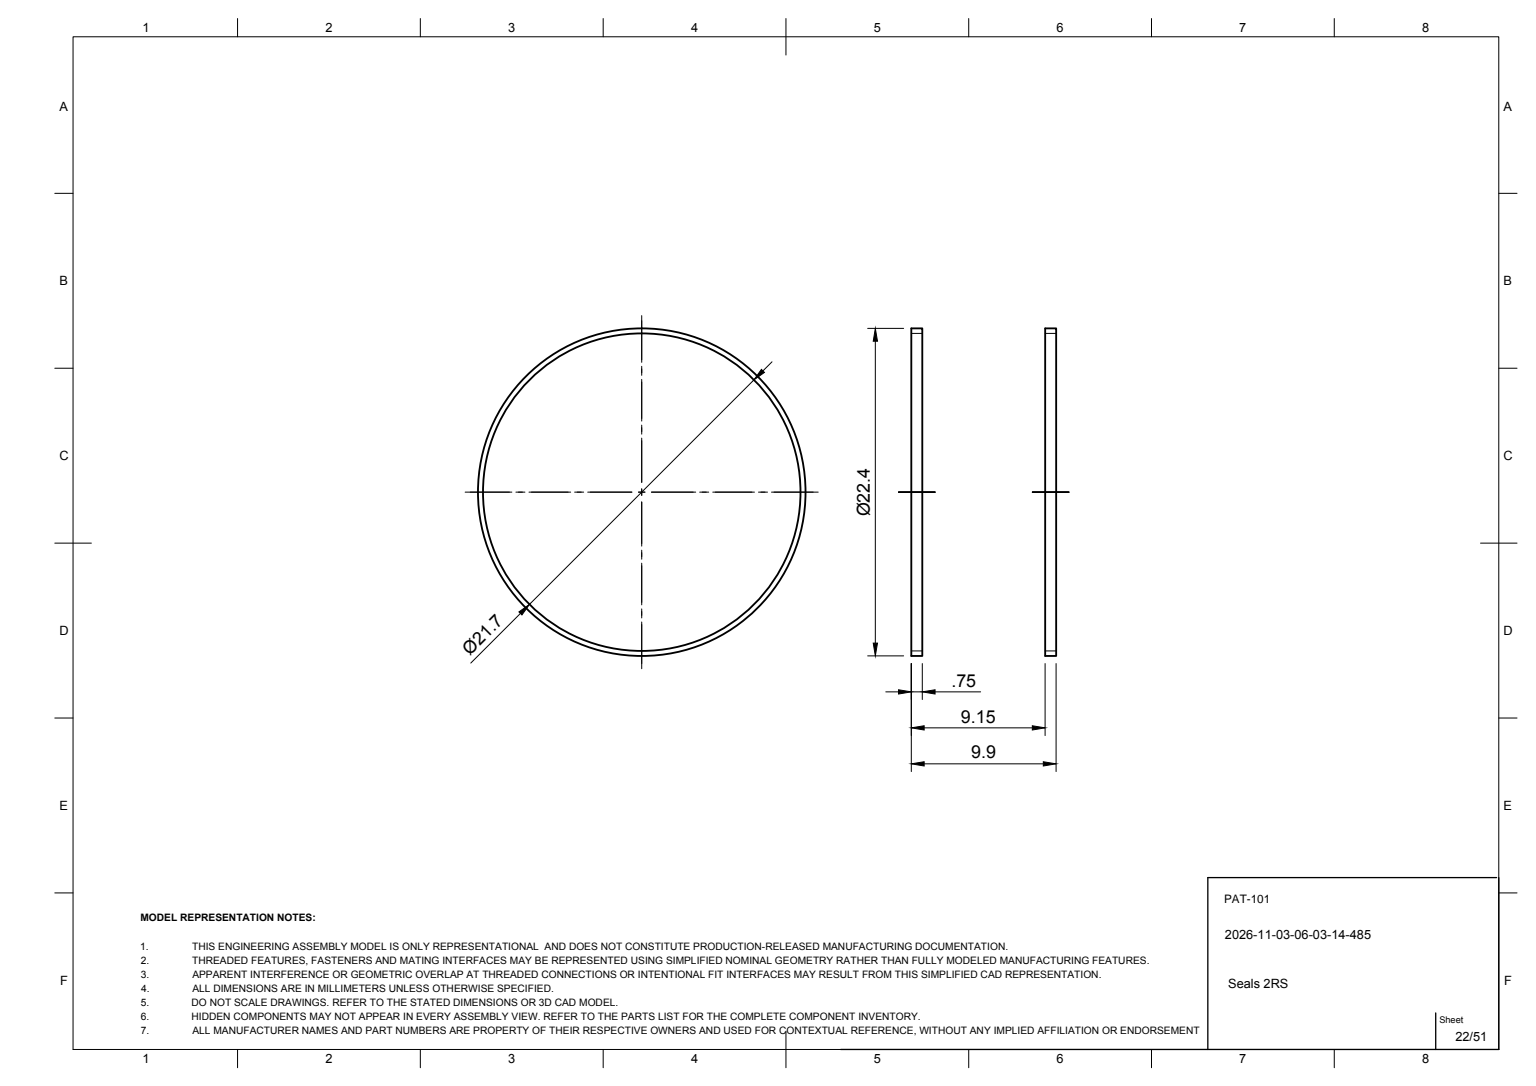
ISO-10303-21;
HEADER;
/* Generated by software containing ST-Developer
 * from STEP Tools, Inc. (www.steptools.com) 
 */

FILE_DESCRIPTION(
/* description */ ('Spur gear reduction stage 2-1 on bearing plates'),
/* implementation_level */ '2;1');

FILE_NAME(
/* name */ 'Seals 2RS.step',
/* time_stamp */ '2026-10-28T03:22:07-07:00',
/* author */ (''),
/* organization */ (''),
/* preprocessor_version */ 'ST-DEVELOPER v20.2',
/* originating_system */ 'Autodesk Translation Framework v15.17.0.0',
/* authorisation */ '');

FILE_SCHEMA (('AUTOMOTIVE_DESIGN { 1 0 10303 214 3 1 1 }'));
ENDSEC;

DATA;
#10=MECHANICAL_DESIGN_GEOMETRIC_PRESENTATION_REPRESENTATION('',(#970,#971),#53909);
#878=SHAPE_REPRESENTATION_RELATIONSHIP('SRR','None',#54106,#921);
#921=ADVANCED_BREP_SHAPE_REPRESENTATION('',(#1026,#1027),#53880);
#970=STYLED_ITEM('',(#54397),#1026);
#971=STYLED_ITEM('',(#54397),#1027);
#1026=MANIFOLD_SOLID_BREP('Body1',#11296);
#1027=MANIFOLD_SOLID_BREP('Body2',#11297);
#1183=FACE_BOUND('',#2479,.T.);
#1184=FACE_BOUND('',#2482,.T.);
#1185=FACE_BOUND('',#2485,.T.);
#1186=FACE_BOUND('',#2488,.T.);
#1326=PLANE('',#12260);
#1327=PLANE('',#12265);
#1328=PLANE('',#12268);
#1329=PLANE('',#12273);
#1707=FACE_OUTER_BOUND('',#2478,.T.);
#1708=FACE_OUTER_BOUND('',#2480,.T.);
#1709=FACE_OUTER_BOUND('',#2481,.T.);
#1710=FACE_OUTER_BOUND('',#2483,.T.);
#1711=FACE_OUTER_BOUND('',#2484,.T.);
#1712=FACE_OUTER_BOUND('',#2486,.T.);
#1713=FACE_OUTER_BOUND('',#2487,.T.);
#1714=FACE_OUTER_BOUND('',#2489,.T.);
#2478=EDGE_LOOP('',(#8182));
#2479=EDGE_LOOP('',(#8183));
#2480=EDGE_LOOP('',(#8184,#8185,#8186,#8187));
#2481=EDGE_LOOP('',(#8188));
#2482=EDGE_LOOP('',(#8189));
#2483=EDGE_LOOP('',(#8190,#8191,#8192,#8193));
#2484=EDGE_LOOP('',(#8194));
#2485=EDGE_LOOP('',(#8195));
#2486=EDGE_LOOP('',(#8196,#8197,#8198,#8199));
#2487=EDGE_LOOP('',(#8200));
#2488=EDGE_LOOP('',(#8201));
#2489=EDGE_LOOP('',(#8202,#8203,#8204,#8205));
#3149=LINE('',#17199,#3790);
#3150=LINE('',#17204,#3791);
#3151=LINE('',#17213,#3792);
#3152=LINE('',#17218,#3793);
#3790=VECTOR('',#14072,1.119765);
#3791=VECTOR('',#14079,1.085235);
#3792=VECTOR('',#14090,1.119765);
#3793=VECTOR('',#14097,1.085235);
#4488=CIRCLE('',#12261,1.119765);
#4489=CIRCLE('',#12262,1.085235);
#4490=CIRCLE('',#12264,1.119765);
#4491=CIRCLE('',#12266,1.085235);
#4492=CIRCLE('',#12269,1.119765);
#4493=CIRCLE('',#12270,1.085235);
#4494=CIRCLE('',#12272,1.119765);
#4495=CIRCLE('',#12274,1.085235);
#5066=VERTEX_POINT('',#17192);
#5067=VERTEX_POINT('',#17194);
#5068=VERTEX_POINT('',#17197);
#5069=VERTEX_POINT('',#17201);
#5070=VERTEX_POINT('',#17206);
#5071=VERTEX_POINT('',#17208);
#5072=VERTEX_POINT('',#17211);
#5073=VERTEX_POINT('',#17215);
#6233=EDGE_CURVE('',#5066,#5066,#4488,.T.);
#6234=EDGE_CURVE('',#5067,#5067,#4489,.T.);
#6235=EDGE_CURVE('',#5068,#5068,#4490,.T.);
#6236=EDGE_CURVE('',#5068,#5066,#3149,.T.);
#6237=EDGE_CURVE('',#5069,#5069,#4491,.T.);
#6238=EDGE_CURVE('',#5069,#5067,#3150,.T.);
#6239=EDGE_CURVE('',#5070,#5070,#4492,.T.);
#6240=EDGE_CURVE('',#5071,#5071,#4493,.T.);
#6241=EDGE_CURVE('',#5072,#5072,#4494,.T.);
#6242=EDGE_CURVE('',#5072,#5070,#3151,.T.);
#6243=EDGE_CURVE('',#5073,#5073,#4495,.T.);
#6244=EDGE_CURVE('',#5073,#5071,#3152,.T.);
#8182=ORIENTED_EDGE('',*,*,#6233,.F.);
#8183=ORIENTED_EDGE('',*,*,#6234,.T.);
#8184=ORIENTED_EDGE('',*,*,#6235,.F.);
#8185=ORIENTED_EDGE('',*,*,#6236,.T.);
#8186=ORIENTED_EDGE('',*,*,#6233,.T.);
#8187=ORIENTED_EDGE('',*,*,#6236,.F.);
#8188=ORIENTED_EDGE('',*,*,#6235,.T.);
#8189=ORIENTED_EDGE('',*,*,#6237,.F.);
#8190=ORIENTED_EDGE('',*,*,#6237,.T.);
#8191=ORIENTED_EDGE('',*,*,#6238,.T.);
#8192=ORIENTED_EDGE('',*,*,#6234,.F.);
#8193=ORIENTED_EDGE('',*,*,#6238,.F.);
#8194=ORIENTED_EDGE('',*,*,#6239,.F.);
#8195=ORIENTED_EDGE('',*,*,#6240,.T.);
#8196=ORIENTED_EDGE('',*,*,#6241,.F.);
#8197=ORIENTED_EDGE('',*,*,#6242,.T.);
#8198=ORIENTED_EDGE('',*,*,#6239,.T.);
#8199=ORIENTED_EDGE('',*,*,#6242,.F.);
#8200=ORIENTED_EDGE('',*,*,#6241,.T.);
#8201=ORIENTED_EDGE('',*,*,#6243,.F.);
#8202=ORIENTED_EDGE('',*,*,#6243,.T.);
#8203=ORIENTED_EDGE('',*,*,#6244,.T.);
#8204=ORIENTED_EDGE('',*,*,#6240,.F.);
#8205=ORIENTED_EDGE('',*,*,#6244,.F.);
#10508=CYLINDRICAL_SURFACE('',#12263,1.119765);
#10509=CYLINDRICAL_SURFACE('',#12267,1.085235);
#10510=CYLINDRICAL_SURFACE('',#12271,1.119765);
#10511=CYLINDRICAL_SURFACE('',#12275,1.085235);
#10827=ADVANCED_FACE('',(#1707,#1183),#1326,.T.);
#10828=ADVANCED_FACE('',(#1708),#10508,.T.);
#10829=ADVANCED_FACE('',(#1709,#1184),#1327,.T.);
#10830=ADVANCED_FACE('',(#1710),#10509,.F.);
#10831=ADVANCED_FACE('',(#1711,#1185),#1328,.T.);
#10832=ADVANCED_FACE('',(#1712),#10510,.T.);
#10833=ADVANCED_FACE('',(#1713,#1186),#1329,.T.);
#10834=ADVANCED_FACE('',(#1714),#10511,.F.);
#11296=CLOSED_SHELL('',(#10827,#10828,#10829,#10830));
#11297=CLOSED_SHELL('',(#10831,#10832,#10833,#10834));
#12259=AXIS2_PLACEMENT_3D('',#17190,#14060,#14061);
#12260=AXIS2_PLACEMENT_3D('',#17191,#14062,#14063);
#12261=AXIS2_PLACEMENT_3D('',#17193,#14064,#14065);
#12262=AXIS2_PLACEMENT_3D('',#17195,#14066,#14067);
#12263=AXIS2_PLACEMENT_3D('',#17196,#14068,#14069);
#12264=AXIS2_PLACEMENT_3D('',#17198,#14070,#14071);
#12265=AXIS2_PLACEMENT_3D('',#17200,#14073,#14074);
#12266=AXIS2_PLACEMENT_3D('',#17202,#14075,#14076);
#12267=AXIS2_PLACEMENT_3D('',#17203,#14077,#14078);
#12268=AXIS2_PLACEMENT_3D('',#17205,#14080,#14081);
#12269=AXIS2_PLACEMENT_3D('',#17207,#14082,#14083);
#12270=AXIS2_PLACEMENT_3D('',#17209,#14084,#14085);
#12271=AXIS2_PLACEMENT_3D('',#17210,#14086,#14087);
#12272=AXIS2_PLACEMENT_3D('',#17212,#14088,#14089);
#12273=AXIS2_PLACEMENT_3D('',#17214,#14091,#14092);
#12274=AXIS2_PLACEMENT_3D('',#17216,#14093,#14094);
#12275=AXIS2_PLACEMENT_3D('',#17217,#14095,#14096);
#14060=DIRECTION('axis',(0.,0.,1.));
#14061=DIRECTION('refdir',(1.,0.,0.));
#14062=DIRECTION('center_axis',(0.,1.,0.));
#14063=DIRECTION('ref_axis',(0.,0.,1.));
#14064=DIRECTION('center_axis',(0.,-1.,0.));
#14065=DIRECTION('ref_axis',(1.,0.,0.));
#14066=DIRECTION('center_axis',(0.,-1.,0.));
#14067=DIRECTION('ref_axis',(1.,0.,0.));
#14068=DIRECTION('center_axis',(0.,-1.,0.));
#14069=DIRECTION('ref_axis',(1.,0.,0.));
#14070=DIRECTION('center_axis',(0.,-1.,0.));
#14071=DIRECTION('ref_axis',(1.,0.,0.));
#14072=DIRECTION('',(0.,1.,0.));
#14073=DIRECTION('center_axis',(0.,-1.,0.));
#14074=DIRECTION('ref_axis',(0.,0.,-1.));
#14075=DIRECTION('center_axis',(0.,-1.,0.));
#14076=DIRECTION('ref_axis',(1.,0.,0.));
#14077=DIRECTION('center_axis',(0.,-1.,0.));
#14078=DIRECTION('ref_axis',(1.,0.,0.));
#14079=DIRECTION('',(0.,1.,0.));
#14080=DIRECTION('center_axis',(0.,1.,0.));
#14081=DIRECTION('ref_axis',(0.,0.,1.));
#14082=DIRECTION('center_axis',(0.,-1.,0.));
#14083=DIRECTION('ref_axis',(1.,0.,0.));
#14084=DIRECTION('center_axis',(0.,-1.,0.));
#14085=DIRECTION('ref_axis',(1.,0.,0.));
#14086=DIRECTION('center_axis',(0.,-1.,0.));
#14087=DIRECTION('ref_axis',(1.,0.,0.));
#14088=DIRECTION('center_axis',(0.,-1.,0.));
#14089=DIRECTION('ref_axis',(1.,0.,0.));
#14090=DIRECTION('',(0.,1.,0.));
#14091=DIRECTION('center_axis',(0.,-1.,0.));
#14092=DIRECTION('ref_axis',(0.,0.,-1.));
#14093=DIRECTION('center_axis',(0.,-1.,0.));
#14094=DIRECTION('ref_axis',(1.,0.,0.));
#14095=DIRECTION('center_axis',(0.,-1.,0.));
#14096=DIRECTION('ref_axis',(1.,0.,0.));
#14097=DIRECTION('',(0.,1.,0.));
#17190=CARTESIAN_POINT('',(0.,0.,0.));
#17191=CARTESIAN_POINT('Origin',(1.119765,0.495,0.));
#17192=CARTESIAN_POINT('',(-1.119765,0.495,-1.37131662304724E-16));
#17193=CARTESIAN_POINT('Origin',(0.,0.495,0.));
#17194=CARTESIAN_POINT('',(-1.085235,0.495,-1.32902956907268E-16));
#17195=CARTESIAN_POINT('Origin',(0.,0.495,0.));
#17196=CARTESIAN_POINT('Origin',(0.,0.4575,0.));
#17197=CARTESIAN_POINT('',(-1.119765,0.42,-1.37131662304724E-16));
#17198=CARTESIAN_POINT('Origin',(0.,0.42,0.));
#17199=CARTESIAN_POINT('',(-1.119765,0.4575,-1.37131662304724E-16));
#17200=CARTESIAN_POINT('Origin',(1.085235,0.42,0.));
#17201=CARTESIAN_POINT('',(-1.085235,0.42,-1.32902956907268E-16));
#17202=CARTESIAN_POINT('Origin',(0.,0.42,0.));
#17203=CARTESIAN_POINT('Origin',(0.,0.4575,0.));
#17204=CARTESIAN_POINT('',(-1.085235,0.4575,-1.32902956907268E-16));
#17205=CARTESIAN_POINT('Origin',(1.119765,-0.42,0.));
#17206=CARTESIAN_POINT('',(-1.119765,-0.42,-1.37131662304724E-16));
#17207=CARTESIAN_POINT('Origin',(0.,-0.42,0.));
#17208=CARTESIAN_POINT('',(-1.085235,-0.42,-1.32902956907268E-16));
#17209=CARTESIAN_POINT('Origin',(0.,-0.42,0.));
#17210=CARTESIAN_POINT('Origin',(0.,-0.4575,0.));
#17211=CARTESIAN_POINT('',(-1.119765,-0.495,-1.37131662304724E-16));
#17212=CARTESIAN_POINT('Origin',(0.,-0.495,0.));
#17213=CARTESIAN_POINT('',(-1.119765,-0.4575,-1.37131662304724E-16));
#17214=CARTESIAN_POINT('Origin',(1.085235,-0.495,0.));
#17215=CARTESIAN_POINT('',(-1.085235,-0.495,-1.32902956907268E-16));
#17216=CARTESIAN_POINT('Origin',(0.,-0.495,0.));
#17217=CARTESIAN_POINT('Origin',(0.,-0.4575,0.));
#17218=CARTESIAN_POINT('',(-1.085235,-0.4575,-1.32902956907268E-16));
#53830=UNCERTAINTY_MEASURE_WITH_UNIT(LENGTH_MEASURE(0.001),#53910,
'DISTANCE_ACCURACY_VALUE',
'Maximum model space distance between geometric entities at asserted c
onnectivities');
#53859=UNCERTAINTY_MEASURE_WITH_UNIT(LENGTH_MEASURE(0.001),#53910,
'DISTANCE_ACCURACY_VALUE',
'Maximum model space distance between geometric entities at asserted c
onnectivities');
#53880=(
GEOMETRIC_REPRESENTATION_CONTEXT(3)
GLOBAL_UNCERTAINTY_ASSIGNED_CONTEXT((#53830))
GLOBAL_UNIT_ASSIGNED_CONTEXT((#53910,#53912,#53913))
REPRESENTATION_CONTEXT('','3D')
);
#53909=(
GEOMETRIC_REPRESENTATION_CONTEXT(3)
GLOBAL_UNCERTAINTY_ASSIGNED_CONTEXT((#53859))
GLOBAL_UNIT_ASSIGNED_CONTEXT((#53910,#53912,#53913))
REPRESENTATION_CONTEXT('','3D')
);
#53910=(
LENGTH_UNIT()
NAMED_UNIT(*)
SI_UNIT(.CENTI.,.METRE.)
);
#53912=(
NAMED_UNIT(*)
PLANE_ANGLE_UNIT()
SI_UNIT($,.RADIAN.)
);
#53913=(
NAMED_UNIT(*)
SI_UNIT($,.STERADIAN.)
SOLID_ANGLE_UNIT()
);
#53934=SHAPE_DEFINITION_REPRESENTATION(#53983,#54106);
#53983=PRODUCT_DEFINITION_SHAPE('',$,#54156);
#54106=SHAPE_REPRESENTATION('',(#12259),#53880);
#54135=PRODUCT_DEFINITION_CONTEXT('part definition',#54284,'design');
#54156=PRODUCT_DEFINITION('Seals 2RS','Seals 2RS',#54205,#54135);
#54205=PRODUCT_DEFINITION_FORMATION('',$,#54306);
#54284=APPLICATION_CONTEXT(
'Core Data for Automotive Mechanical Design Process');
#54285=PRODUCT_CONTEXT('part definition',#54284,'mechanical');
#54306=PRODUCT('Seals 2RS','Seals 2RS','Seals 2RS',(#54285));
#54391=COLOUR_RGB('Grey',0.48,0.52,0.57);
#54392=FILL_AREA_STYLE_COLOUR('',#54391);
#54393=FILL_AREA_STYLE('',(#54392));
#54394=SURFACE_STYLE_FILL_AREA(#54393);
#54395=SURFACE_SIDE_STYLE('',(#54394));
#54396=SURFACE_STYLE_USAGE(.BOTH.,#54395);
#54397=PRESENTATION_STYLE_ASSIGNMENT((#54396));
ENDSEC;
END-ISO-10303-21;
